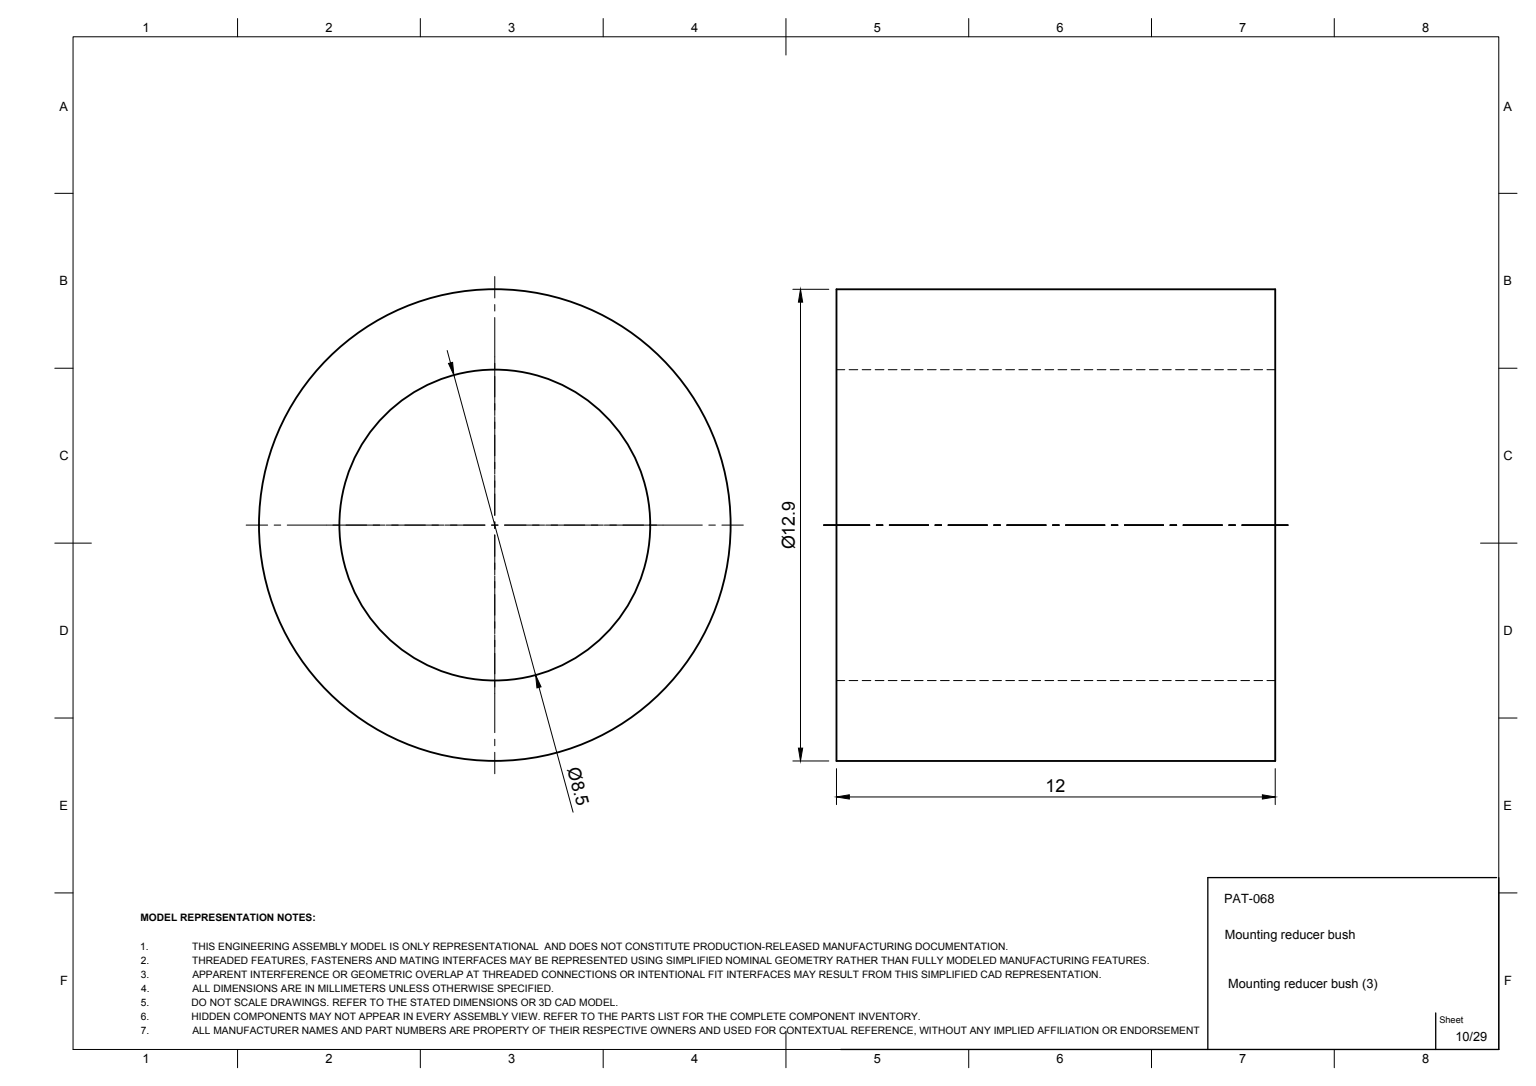
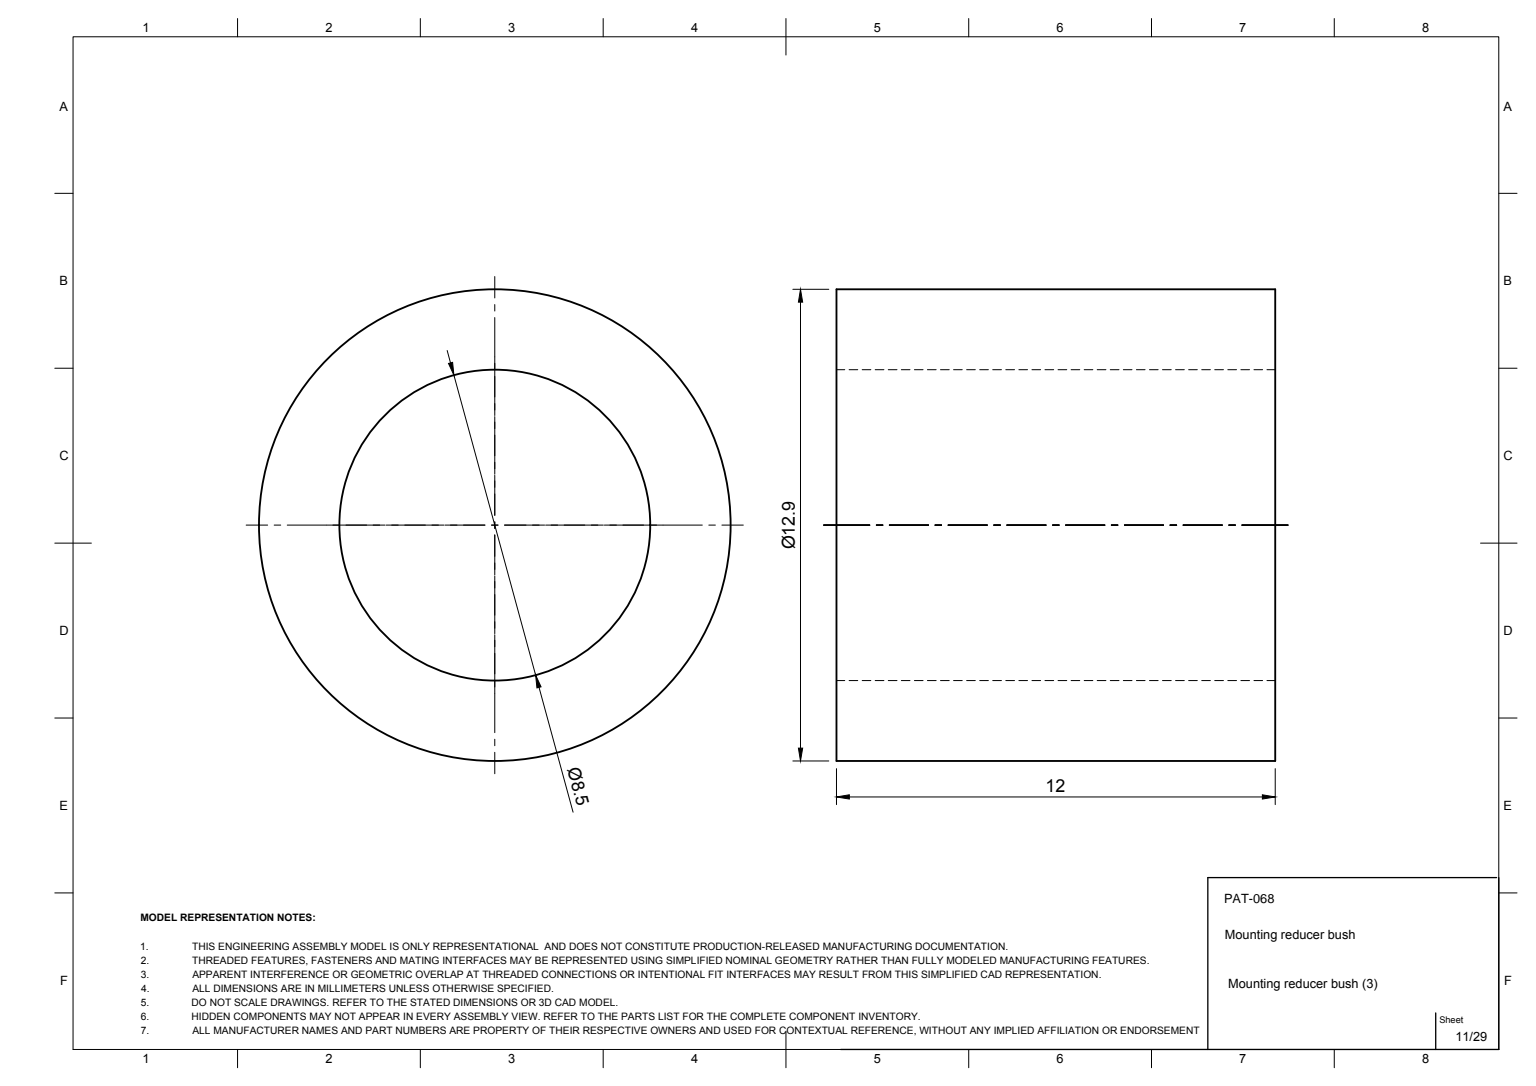
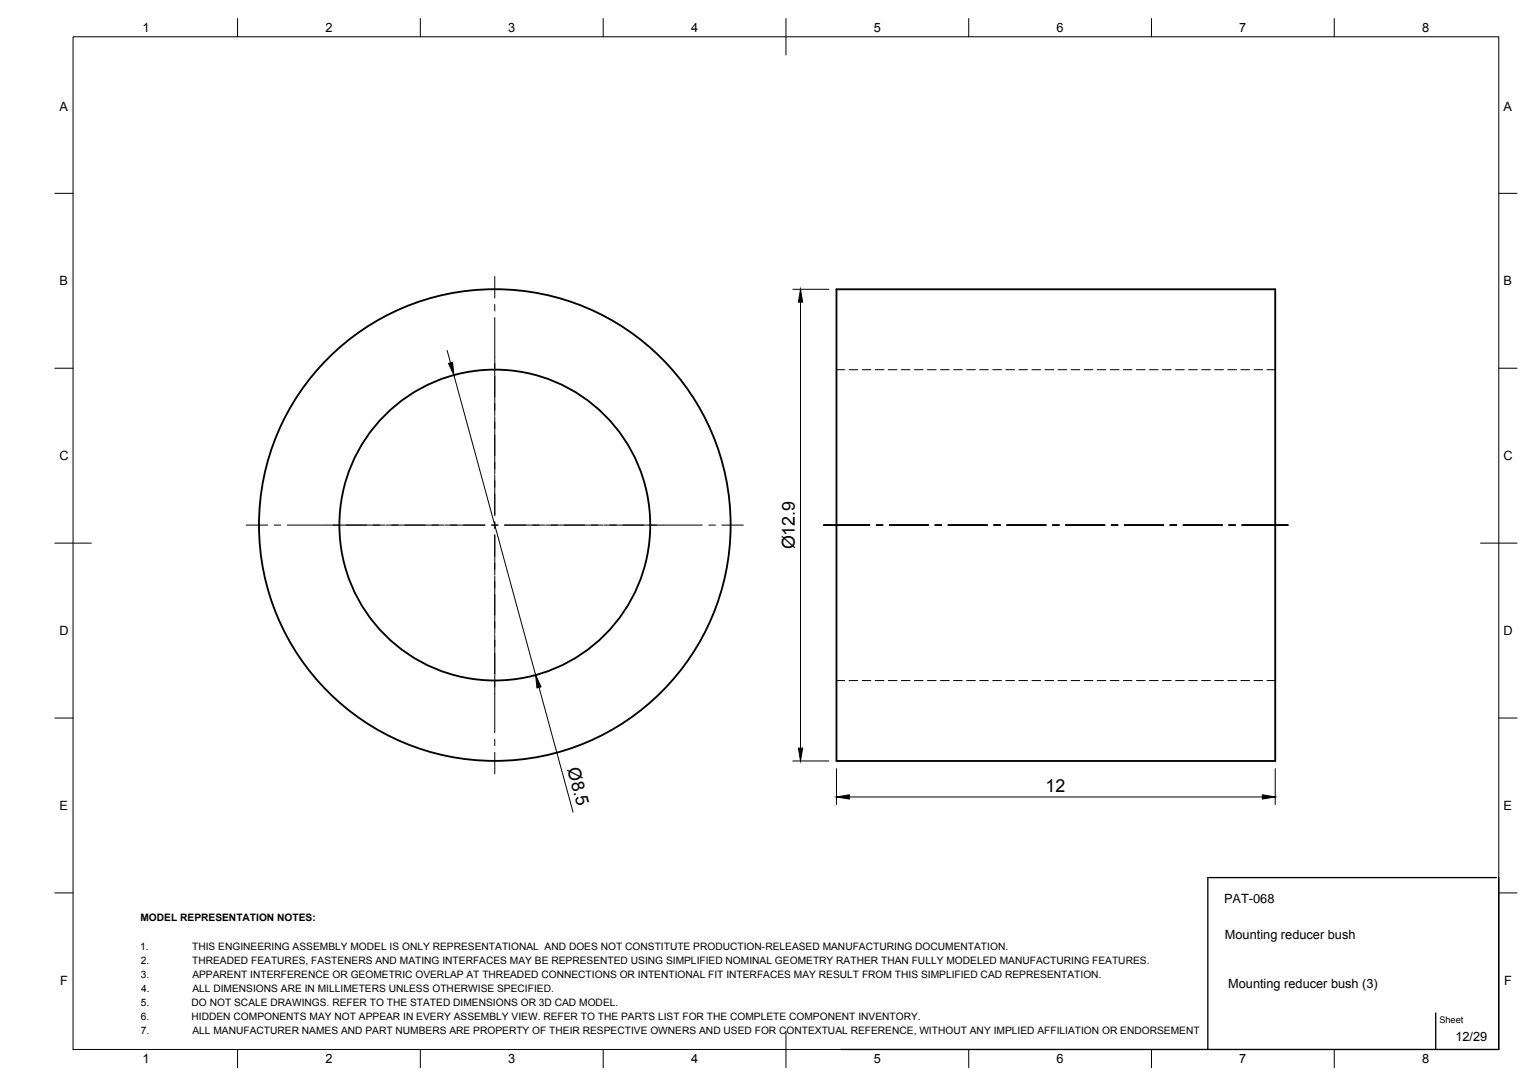
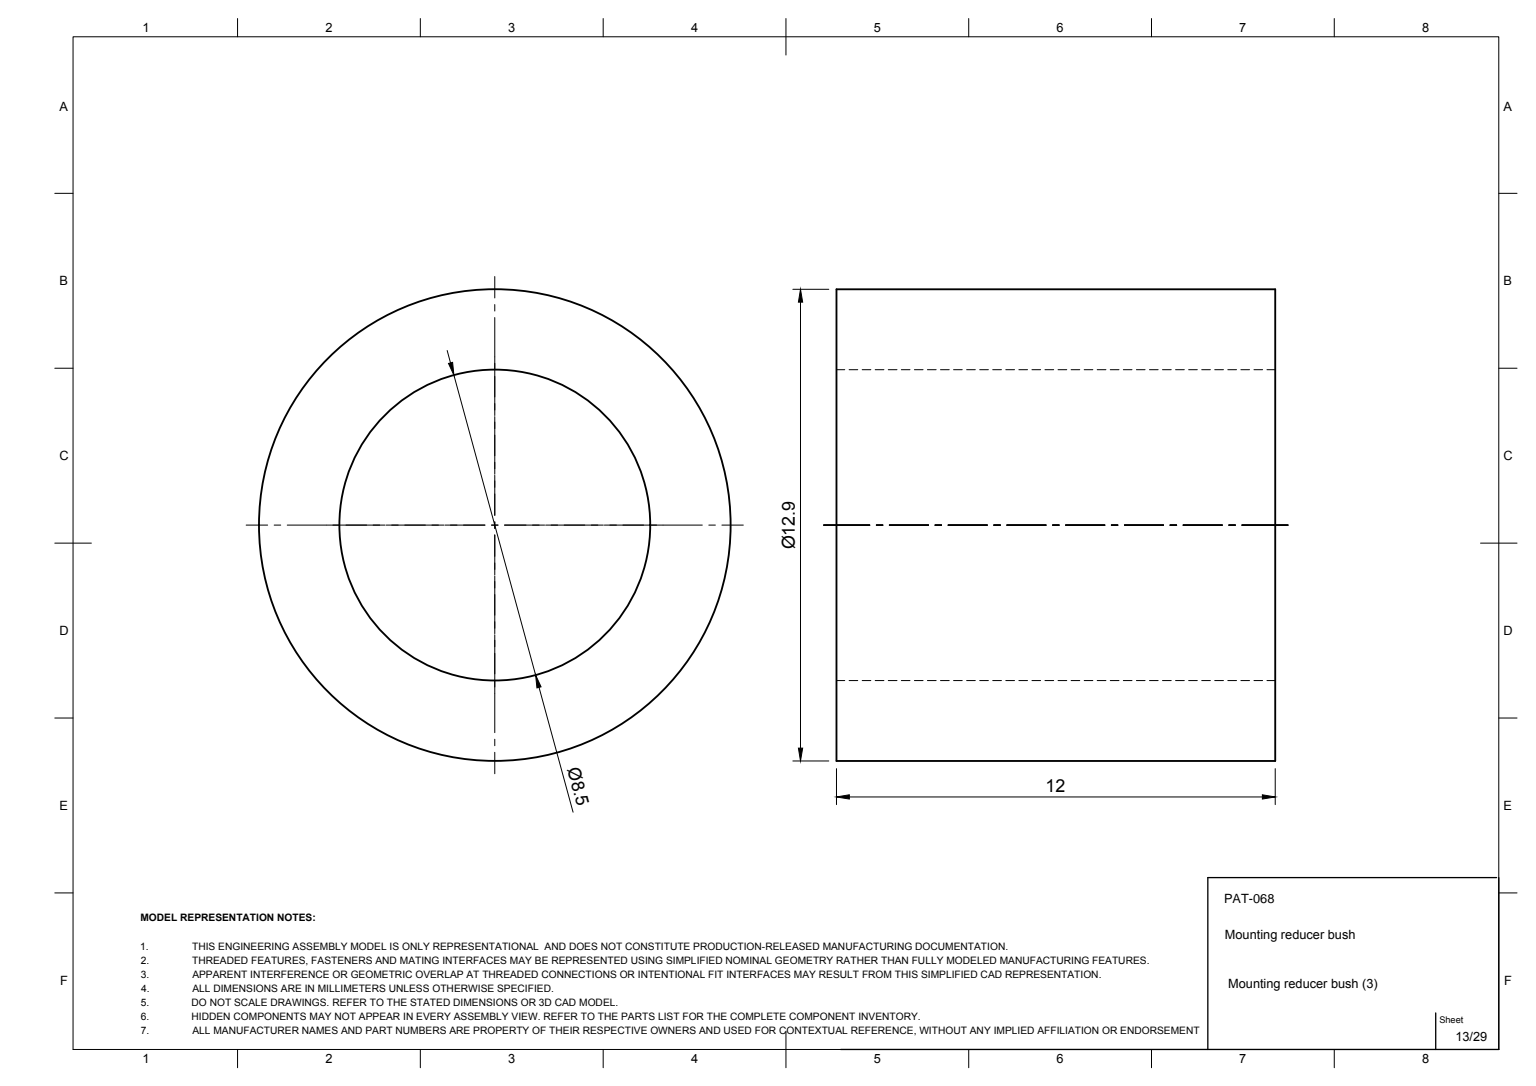
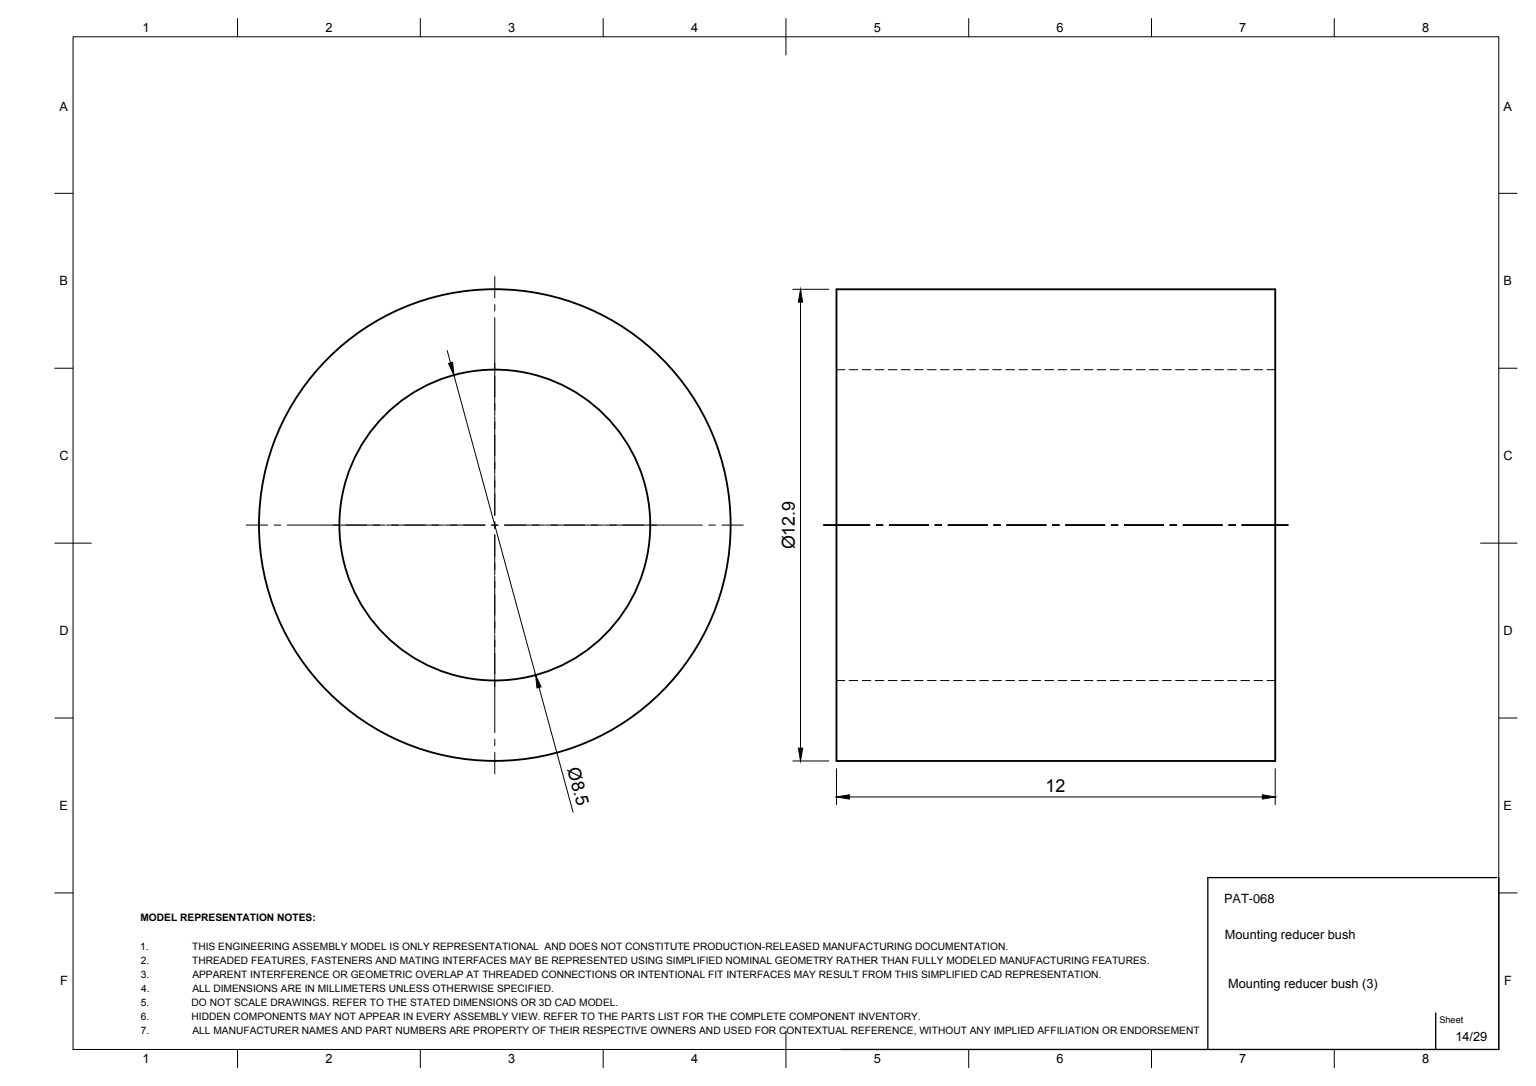
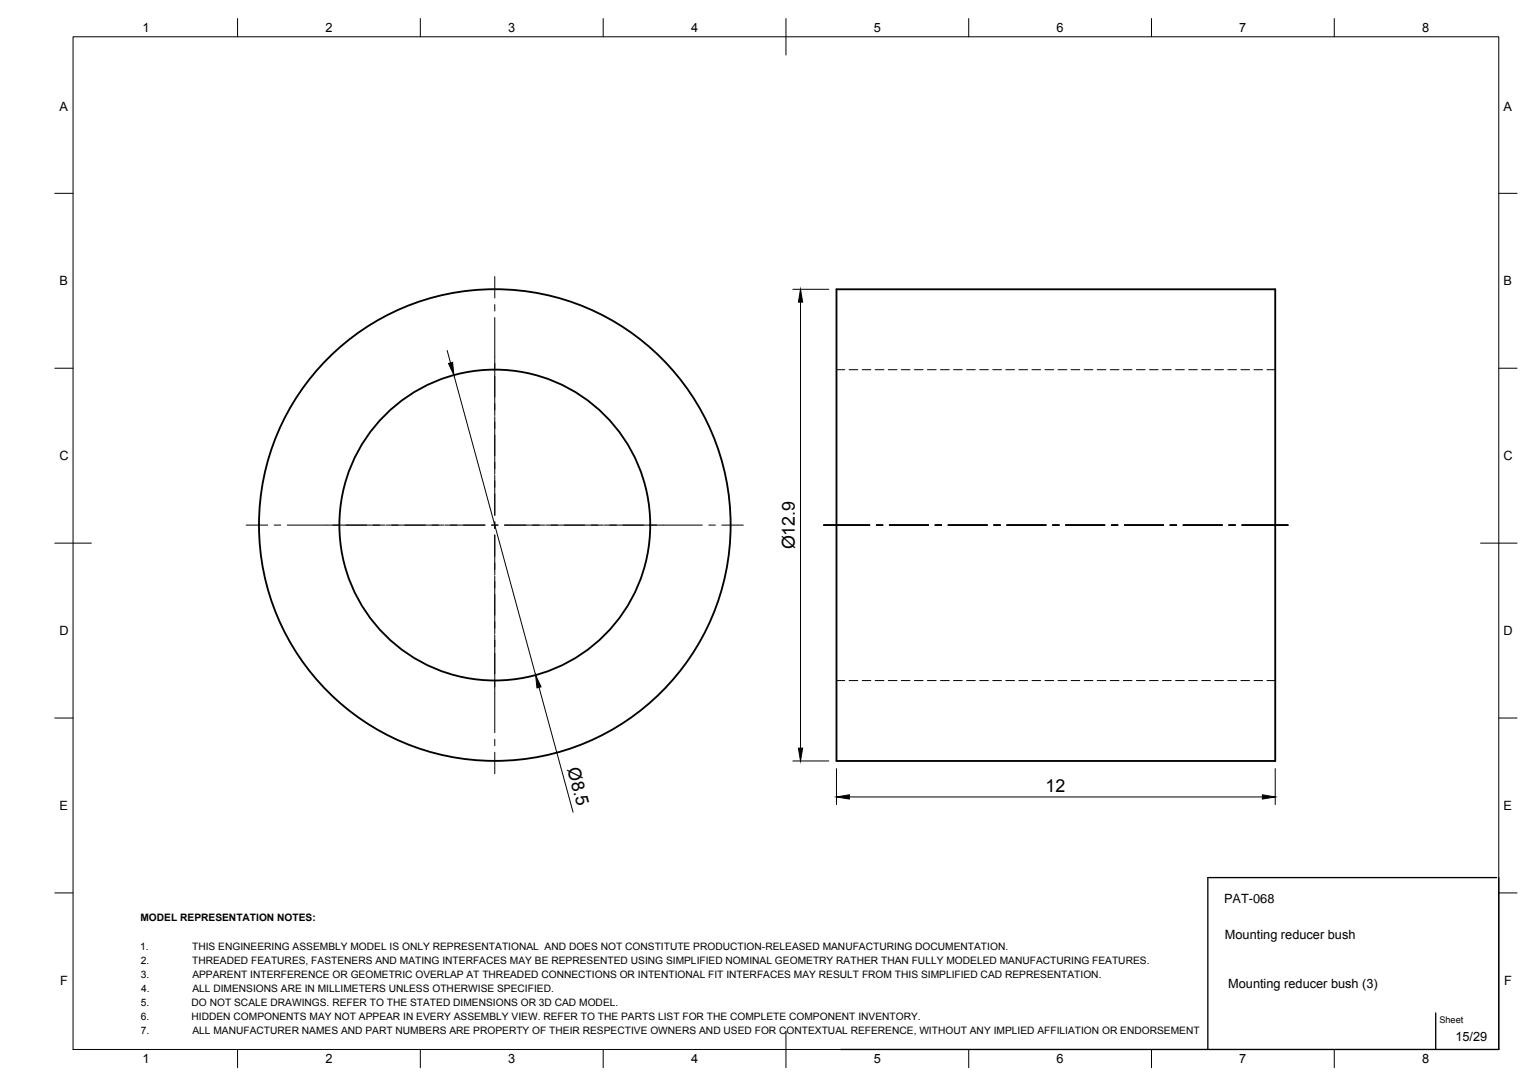
ISO-10303-21;
HEADER;
/* Generated by software containing ST-Developer
 * from STEP Tools, Inc. (www.steptools.com) 
 */

FILE_DESCRIPTION(
/* description */ ('Line shaft on three pillow blocks'),
/* implementation_level */ '2;1');

FILE_NAME(
/* name */ 'Mounting reducer bush.step',
/* time_stamp */ '2026-10-27T10:49:19-07:00',
/* author */ (''),
/* organization */ (''),
/* preprocessor_version */ 'ST-DEVELOPER v20.2',
/* originating_system */ 'Autodesk Translation Framework v15.17.0.0',
/* authorisation */ '');

FILE_SCHEMA (('AUTOMOTIVE_DESIGN { 1 0 10303 214 3 1 1 }'));
ENDSEC;

DATA;
#10=MECHANICAL_DESIGN_GEOMETRIC_PRESENTATION_REPRESENTATION('',(#343),#8377);
#289=SHAPE_REPRESENTATION_RELATIONSHIP('SRR','None',#8504,#316);
#316=ADVANCED_BREP_SHAPE_REPRESENTATION('',(#371),#8353);
#343=STYLED_ITEM('',(#8732),#371);
#371=MANIFOLD_SOLID_BREP('Body1',#4329);
#415=FACE_BOUND('',#981,.T.);
#416=FACE_BOUND('',#983,.T.);
#522=PLANE('',#4743);
#523=PLANE('',#4744);
#702=FACE_OUTER_BOUND('',#978,.T.);
#703=FACE_OUTER_BOUND('',#979,.T.);
#704=FACE_OUTER_BOUND('',#980,.T.);
#705=FACE_OUTER_BOUND('',#982,.T.);
#978=EDGE_LOOP('',(#3153,#3154,#3155,#3156));
#979=EDGE_LOOP('',(#3157,#3158,#3159,#3160));
#980=EDGE_LOOP('',(#3161));
#981=EDGE_LOOP('',(#3162));
#982=EDGE_LOOP('',(#3163));
#983=EDGE_LOOP('',(#3164));
#1329=LINE('',#6695,#1656);
#1330=LINE('',#6701,#1657);
#1656=VECTOR('',#5394,0.425);
#1657=VECTOR('',#5401,0.645);
#1937=CIRCLE('',#4738,0.425);
#1938=CIRCLE('',#4739,0.425);
#1939=CIRCLE('',#4741,0.645);
#1940=CIRCLE('',#4742,0.645);
#2136=VERTEX_POINT('',#6692);
#2137=VERTEX_POINT('',#6694);
#2138=VERTEX_POINT('',#6698);
#2139=VERTEX_POINT('',#6700);
#2525=EDGE_CURVE('',#2136,#2136,#1937,.T.);
#2526=EDGE_CURVE('',#2136,#2137,#1329,.T.);
#2527=EDGE_CURVE('',#2137,#2137,#1938,.T.);
#2528=EDGE_CURVE('',#2138,#2138,#1939,.T.);
#2529=EDGE_CURVE('',#2138,#2139,#1330,.T.);
#2530=EDGE_CURVE('',#2139,#2139,#1940,.T.);
#3153=ORIENTED_EDGE('',*,*,#2525,.F.);
#3154=ORIENTED_EDGE('',*,*,#2526,.T.);
#3155=ORIENTED_EDGE('',*,*,#2527,.T.);
#3156=ORIENTED_EDGE('',*,*,#2526,.F.);
#3157=ORIENTED_EDGE('',*,*,#2528,.F.);
#3158=ORIENTED_EDGE('',*,*,#2529,.T.);
#3159=ORIENTED_EDGE('',*,*,#2530,.T.);
#3160=ORIENTED_EDGE('',*,*,#2529,.F.);
#3161=ORIENTED_EDGE('',*,*,#2528,.T.);
#3162=ORIENTED_EDGE('',*,*,#2525,.T.);
#3163=ORIENTED_EDGE('',*,*,#2530,.F.);
#3164=ORIENTED_EDGE('',*,*,#2527,.F.);
#4015=CYLINDRICAL_SURFACE('',#4737,0.425);
#4016=CYLINDRICAL_SURFACE('',#4740,0.645);
#4120=ADVANCED_FACE('',(#702),#4015,.F.);
#4121=ADVANCED_FACE('',(#703),#4016,.T.);
#4122=ADVANCED_FACE('',(#704,#415),#522,.T.);
#4123=ADVANCED_FACE('',(#705,#416),#523,.F.);
#4329=CLOSED_SHELL('',(#4120,#4121,#4122,#4123));
#4736=AXIS2_PLACEMENT_3D('',#6690,#5388,#5389);
#4737=AXIS2_PLACEMENT_3D('',#6691,#5390,#5391);
#4738=AXIS2_PLACEMENT_3D('',#6693,#5392,#5393);
#4739=AXIS2_PLACEMENT_3D('',#6696,#5395,#5396);
#4740=AXIS2_PLACEMENT_3D('',#6697,#5397,#5398);
#4741=AXIS2_PLACEMENT_3D('',#6699,#5399,#5400);
#4742=AXIS2_PLACEMENT_3D('',#6702,#5402,#5403);
#4743=AXIS2_PLACEMENT_3D('',#6703,#5404,#5405);
#4744=AXIS2_PLACEMENT_3D('',#6704,#5406,#5407);
#5388=DIRECTION('axis',(0.,0.,1.));
#5389=DIRECTION('refdir',(1.,0.,0.));
#5390=DIRECTION('center_axis',(0.,0.,1.));
#5391=DIRECTION('ref_axis',(1.,0.,0.));
#5392=DIRECTION('center_axis',(0.,0.,-1.));
#5393=DIRECTION('ref_axis',(1.,0.,0.));
#5394=DIRECTION('',(0.,0.,-1.));
#5395=DIRECTION('center_axis',(0.,0.,-1.));
#5396=DIRECTION('ref_axis',(1.,0.,0.));
#5397=DIRECTION('center_axis',(0.,0.,1.));
#5398=DIRECTION('ref_axis',(1.,0.,0.));
#5399=DIRECTION('center_axis',(0.,0.,1.));
#5400=DIRECTION('ref_axis',(1.,0.,0.));
#5401=DIRECTION('',(0.,0.,-1.));
#5402=DIRECTION('center_axis',(0.,0.,1.));
#5403=DIRECTION('ref_axis',(1.,0.,0.));
#5404=DIRECTION('center_axis',(0.,0.,1.));
#5405=DIRECTION('ref_axis',(1.,0.,0.));
#5406=DIRECTION('center_axis',(0.,0.,1.));
#5407=DIRECTION('ref_axis',(1.,0.,0.));
#6690=CARTESIAN_POINT('',(0.,0.,0.));
#6691=CARTESIAN_POINT('Origin',(-4.75,0.,1.2));
#6692=CARTESIAN_POINT('',(-5.175,-5.20474889637625E-17,2.4));
#6693=CARTESIAN_POINT('Origin',(-4.75,0.,2.4));
#6694=CARTESIAN_POINT('',(-5.175,-5.20474889637625E-17,1.2));
#6695=CARTESIAN_POINT('',(-5.175,-5.20474889637625E-17,1.2));
#6696=CARTESIAN_POINT('Origin',(-4.75,0.,1.2));
#6697=CARTESIAN_POINT('Origin',(-4.75,0.,1.2));
#6698=CARTESIAN_POINT('',(-5.395,-7.89897185450042E-17,2.4));
#6699=CARTESIAN_POINT('Origin',(-4.75,0.,2.4));
#6700=CARTESIAN_POINT('',(-5.395,-7.89897185450042E-17,1.2));
#6701=CARTESIAN_POINT('',(-5.395,-7.89897185450042E-17,1.2));
#6702=CARTESIAN_POINT('Origin',(-4.75,0.,1.2));
#6703=CARTESIAN_POINT('Origin',(-4.75,0.,2.4));
#6704=CARTESIAN_POINT('Origin',(-4.75,0.,1.2));
#8321=UNCERTAINTY_MEASURE_WITH_UNIT(LENGTH_MEASURE(0.001),#8378,
'DISTANCE_ACCURACY_VALUE',
'Maximum model space distance between geometric entities at asserted c
onnectivities');
#8345=UNCERTAINTY_MEASURE_WITH_UNIT(LENGTH_MEASURE(0.001),#8378,
'DISTANCE_ACCURACY_VALUE',
'Maximum model space distance between geometric entities at asserted c
onnectivities');
#8353=(
GEOMETRIC_REPRESENTATION_CONTEXT(3)
GLOBAL_UNCERTAINTY_ASSIGNED_CONTEXT((#8321))
GLOBAL_UNIT_ASSIGNED_CONTEXT((#8378,#8380,#8381))
REPRESENTATION_CONTEXT('','3D')
);
#8377=(
GEOMETRIC_REPRESENTATION_CONTEXT(3)
GLOBAL_UNCERTAINTY_ASSIGNED_CONTEXT((#8345))
GLOBAL_UNIT_ASSIGNED_CONTEXT((#8378,#8380,#8381))
REPRESENTATION_CONTEXT('','3D')
);
#8378=(
LENGTH_UNIT()
NAMED_UNIT(*)
SI_UNIT(.CENTI.,.METRE.)
);
#8380=(
NAMED_UNIT(*)
PLANE_ANGLE_UNIT()
SI_UNIT($,.RADIAN.)
);
#8381=(
NAMED_UNIT(*)
SI_UNIT($,.STERADIAN.)
SOLID_ANGLE_UNIT()
);
#8389=SHAPE_DEFINITION_REPRESENTATION(#8420,#8504);
#8420=PRODUCT_DEFINITION_SHAPE('',$,#8536);
#8504=SHAPE_REPRESENTATION('',(#4736),#8353);
#8528=PRODUCT_DEFINITION_CONTEXT('part definition',#8623,'design');
#8536=PRODUCT_DEFINITION('Mounting reducer bush',
'Mounting reducer bush',#8567,#8528);
#8567=PRODUCT_DEFINITION_FORMATION('',$,#8632);
#8623=APPLICATION_CONTEXT(
'Core Data for Automotive Mechanical Design Process');
#8624=PRODUCT_CONTEXT('part definition',#8623,'mechanical');
#8632=PRODUCT('Mounting reducer bush','Mounting reducer bush',
'Mounting reducer bush',(#8624));
#8726=COLOUR_RGB('Off White',0.89,0.88,0.83);
#8727=FILL_AREA_STYLE_COLOUR('',#8726);
#8728=FILL_AREA_STYLE('',(#8727));
#8729=SURFACE_STYLE_FILL_AREA(#8728);
#8730=SURFACE_SIDE_STYLE('',(#8729));
#8731=SURFACE_STYLE_USAGE(.BOTH.,#8730);
#8732=PRESENTATION_STYLE_ASSIGNMENT((#8731));
ENDSEC;
END-ISO-10303-21;
